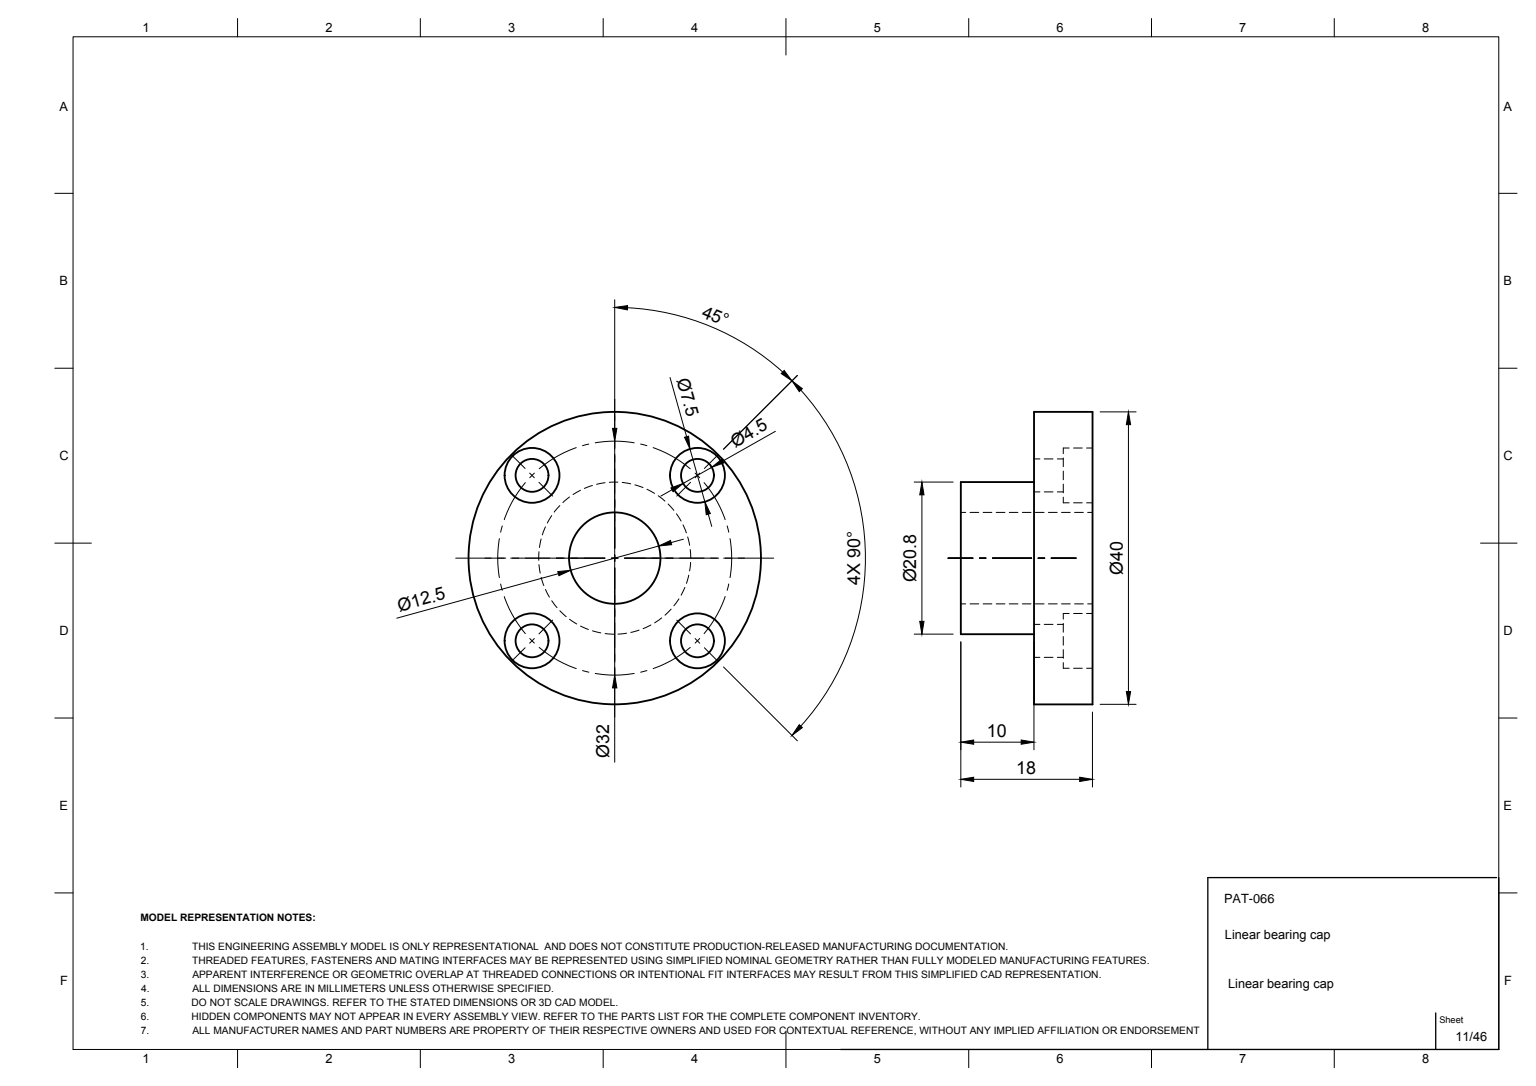
ISO-10303-21;
HEADER;
/* Generated by software containing ST-Developer
 * from STEP Tools, Inc. (www.steptools.com) 
 */

FILE_DESCRIPTION(
/* description */ ('Lever-operated bar clamp (toggle)'),
/* implementation_level */ '2;1');

FILE_NAME(
/* name */ 'Linear bearing cap.step',
/* time_stamp */ '2026-10-28T03:25:02-07:00',
/* author */ (''),
/* organization */ (''),
/* preprocessor_version */ 'ST-DEVELOPER v20.2',
/* originating_system */ 'Autodesk Translation Framework v15.17.0.0',
/* authorisation */ '');

FILE_SCHEMA (('AUTOMOTIVE_DESIGN { 1 0 10303 214 3 1 1 }'));
ENDSEC;

DATA;
#10=MECHANICAL_DESIGN_GEOMETRIC_PRESENTATION_REPRESENTATION('',(#416),#12413);
#340=SHAPE_REPRESENTATION_RELATIONSHIP('SRR','None',#12579,#378);
#378=ADVANCED_BREP_SHAPE_REPRESENTATION('',(#463),#12376);
#416=STYLED_ITEM('',(#12869),#463);
#463=MANIFOLD_SOLID_BREP('Body1',#6575);
#566=FACE_BOUND('',#1446,.T.);
#567=FACE_BOUND('',#1449,.T.);
#568=FACE_BOUND('',#1452,.T.);
#569=FACE_BOUND('',#1455,.T.);
#570=FACE_BOUND('',#1462,.T.);
#571=FACE_BOUND('',#1466,.T.);
#572=FACE_BOUND('',#1467,.T.);
#573=FACE_BOUND('',#1468,.T.);
#574=FACE_BOUND('',#1469,.T.);
#575=FACE_BOUND('',#1470,.T.);
#576=FACE_BOUND('',#1472,.T.);
#577=FACE_BOUND('',#1473,.T.);
#578=FACE_BOUND('',#1474,.T.);
#579=FACE_BOUND('',#1475,.T.);
#580=FACE_BOUND('',#1476,.T.);
#695=PLANE('',#7215);
#696=PLANE('',#7220);
#697=PLANE('',#7225);
#698=PLANE('',#7230);
#699=PLANE('',#7243);
#700=PLANE('',#7250);
#701=PLANE('',#7251);
#972=FACE_OUTER_BOUND('',#1444,.T.);
#973=FACE_OUTER_BOUND('',#1445,.T.);
#974=FACE_OUTER_BOUND('',#1447,.T.);
#975=FACE_OUTER_BOUND('',#1448,.T.);
#976=FACE_OUTER_BOUND('',#1450,.T.);
#977=FACE_OUTER_BOUND('',#1451,.T.);
#978=FACE_OUTER_BOUND('',#1453,.T.);
#979=FACE_OUTER_BOUND('',#1454,.T.);
#980=FACE_OUTER_BOUND('',#1456,.T.);
#981=FACE_OUTER_BOUND('',#1457,.T.);
#982=FACE_OUTER_BOUND('',#1458,.T.);
#983=FACE_OUTER_BOUND('',#1459,.T.);
#984=FACE_OUTER_BOUND('',#1460,.T.);
#985=FACE_OUTER_BOUND('',#1461,.T.);
#986=FACE_OUTER_BOUND('',#1463,.T.);
#987=FACE_OUTER_BOUND('',#1464,.T.);
#988=FACE_OUTER_BOUND('',#1465,.T.);
#989=FACE_OUTER_BOUND('',#1471,.T.);
#1444=EDGE_LOOP('',(#4805,#4806,#4807,#4808));
#1445=EDGE_LOOP('',(#4809));
#1446=EDGE_LOOP('',(#4810));
#1447=EDGE_LOOP('',(#4811,#4812,#4813,#4814));
#1448=EDGE_LOOP('',(#4815));
#1449=EDGE_LOOP('',(#4816));
#1450=EDGE_LOOP('',(#4817,#4818,#4819,#4820));
#1451=EDGE_LOOP('',(#4821));
#1452=EDGE_LOOP('',(#4822));
#1453=EDGE_LOOP('',(#4823,#4824,#4825,#4826));
#1454=EDGE_LOOP('',(#4827));
#1455=EDGE_LOOP('',(#4828));
#1456=EDGE_LOOP('',(#4829,#4830,#4831,#4832));
#1457=EDGE_LOOP('',(#4833,#4834,#4835,#4836));
#1458=EDGE_LOOP('',(#4837,#4838,#4839,#4840));
#1459=EDGE_LOOP('',(#4841,#4842,#4843,#4844));
#1460=EDGE_LOOP('',(#4845,#4846,#4847,#4848));
#1461=EDGE_LOOP('',(#4849));
#1462=EDGE_LOOP('',(#4850));
#1463=EDGE_LOOP('',(#4851,#4852,#4853,#4854));
#1464=EDGE_LOOP('',(#4855,#4856,#4857,#4858));
#1465=EDGE_LOOP('',(#4859));
#1466=EDGE_LOOP('',(#4860));
#1467=EDGE_LOOP('',(#4861));
#1468=EDGE_LOOP('',(#4862));
#1469=EDGE_LOOP('',(#4863));
#1470=EDGE_LOOP('',(#4864));
#1471=EDGE_LOOP('',(#4865));
#1472=EDGE_LOOP('',(#4866));
#1473=EDGE_LOOP('',(#4867));
#1474=EDGE_LOOP('',(#4868));
#1475=EDGE_LOOP('',(#4869));
#1476=EDGE_LOOP('',(#4870));
#1963=LINE('',#10462,#2404);
#1964=LINE('',#10471,#2405);
#1965=LINE('',#10480,#2406);
#1966=LINE('',#10489,#2407);
#1967=LINE('',#10497,#2408);
#1968=LINE('',#10501,#2409);
#1969=LINE('',#10505,#2410);
#1970=LINE('',#10509,#2411);
#1971=LINE('',#10514,#2412);
#1972=LINE('',#10522,#2413);
#1973=LINE('',#10527,#2414);
#2404=VECTOR('',#8356,0.375);
#2405=VECTOR('',#8367,0.375);
#2406=VECTOR('',#8378,0.375);
#2407=VECTOR('',#8389,0.375);
#2408=VECTOR('',#8400,0.225);
#2409=VECTOR('',#8405,0.225);
#2410=VECTOR('',#8410,0.225);
#2411=VECTOR('',#8415,0.225);
#2412=VECTOR('',#8420,1.04);
#2413=VECTOR('',#8431,0.625);
#2414=VECTOR('',#8436,2.);
#2813=CIRCLE('',#7213,0.375);
#2814=CIRCLE('',#7214,0.375);
#2815=CIRCLE('',#7216,0.225);
#2816=CIRCLE('',#7218,0.375);
#2817=CIRCLE('',#7219,0.375);
#2818=CIRCLE('',#7221,0.225);
#2819=CIRCLE('',#7223,0.375);
#2820=CIRCLE('',#7224,0.375);
#2821=CIRCLE('',#7226,0.225);
#2822=CIRCLE('',#7228,0.375);
#2823=CIRCLE('',#7229,0.375);
#2824=CIRCLE('',#7231,0.225);
#2825=CIRCLE('',#7233,0.225);
#2826=CIRCLE('',#7235,0.225);
#2827=CIRCLE('',#7237,0.225);
#2828=CIRCLE('',#7239,0.225);
#2829=CIRCLE('',#7241,1.04);
#2830=CIRCLE('',#7242,1.04);
#2831=CIRCLE('',#7244,0.625);
#2832=CIRCLE('',#7246,0.625);
#2833=CIRCLE('',#7248,2.);
#2834=CIRCLE('',#7249,2.);
#3202=VERTEX_POINT('',#10459);
#3203=VERTEX_POINT('',#10461);
#3204=VERTEX_POINT('',#10465);
#3205=VERTEX_POINT('',#10468);
#3206=VERTEX_POINT('',#10470);
#3207=VERTEX_POINT('',#10474);
#3208=VERTEX_POINT('',#10477);
#3209=VERTEX_POINT('',#10479);
#3210=VERTEX_POINT('',#10483);
#3211=VERTEX_POINT('',#10486);
#3212=VERTEX_POINT('',#10488);
#3213=VERTEX_POINT('',#10492);
#3214=VERTEX_POINT('',#10495);
#3215=VERTEX_POINT('',#10499);
#3216=VERTEX_POINT('',#10503);
#3217=VERTEX_POINT('',#10507);
#3218=VERTEX_POINT('',#10511);
#3219=VERTEX_POINT('',#10513);
#3220=VERTEX_POINT('',#10517);
#3221=VERTEX_POINT('',#10520);
#3222=VERTEX_POINT('',#10524);
#3223=VERTEX_POINT('',#10526);
#3807=EDGE_CURVE('',#3202,#3202,#2813,.T.);
#3808=EDGE_CURVE('',#3202,#3203,#1963,.T.);
#3809=EDGE_CURVE('',#3203,#3203,#2814,.T.);
#3810=EDGE_CURVE('',#3204,#3204,#2815,.T.);
#3811=EDGE_CURVE('',#3205,#3205,#2816,.T.);
#3812=EDGE_CURVE('',#3205,#3206,#1964,.T.);
#3813=EDGE_CURVE('',#3206,#3206,#2817,.T.);
#3814=EDGE_CURVE('',#3207,#3207,#2818,.T.);
#3815=EDGE_CURVE('',#3208,#3208,#2819,.T.);
#3816=EDGE_CURVE('',#3208,#3209,#1965,.T.);
#3817=EDGE_CURVE('',#3209,#3209,#2820,.T.);
#3818=EDGE_CURVE('',#3210,#3210,#2821,.T.);
#3819=EDGE_CURVE('',#3211,#3211,#2822,.T.);
#3820=EDGE_CURVE('',#3211,#3212,#1966,.T.);
#3821=EDGE_CURVE('',#3212,#3212,#2823,.T.);
#3822=EDGE_CURVE('',#3213,#3213,#2824,.T.);
#3823=EDGE_CURVE('',#3214,#3214,#2825,.T.);
#3824=EDGE_CURVE('',#3214,#3204,#1967,.T.);
#3825=EDGE_CURVE('',#3215,#3215,#2826,.T.);
#3826=EDGE_CURVE('',#3215,#3207,#1968,.T.);
#3827=EDGE_CURVE('',#3216,#3216,#2827,.T.);
#3828=EDGE_CURVE('',#3216,#3210,#1969,.T.);
#3829=EDGE_CURVE('',#3217,#3217,#2828,.T.);
#3830=EDGE_CURVE('',#3217,#3213,#1970,.T.);
#3831=EDGE_CURVE('',#3218,#3218,#2829,.T.);
#3832=EDGE_CURVE('',#3218,#3219,#1971,.T.);
#3833=EDGE_CURVE('',#3219,#3219,#2830,.T.);
#3834=EDGE_CURVE('',#3220,#3220,#2831,.T.);
#3835=EDGE_CURVE('',#3221,#3221,#2832,.T.);
#3836=EDGE_CURVE('',#3221,#3220,#1972,.T.);
#3837=EDGE_CURVE('',#3222,#3222,#2833,.T.);
#3838=EDGE_CURVE('',#3222,#3223,#1973,.T.);
#3839=EDGE_CURVE('',#3223,#3223,#2834,.T.);
#4805=ORIENTED_EDGE('',*,*,#3807,.F.);
#4806=ORIENTED_EDGE('',*,*,#3808,.T.);
#4807=ORIENTED_EDGE('',*,*,#3809,.F.);
#4808=ORIENTED_EDGE('',*,*,#3808,.F.);
#4809=ORIENTED_EDGE('',*,*,#3807,.T.);
#4810=ORIENTED_EDGE('',*,*,#3810,.F.);
#4811=ORIENTED_EDGE('',*,*,#3811,.F.);
#4812=ORIENTED_EDGE('',*,*,#3812,.T.);
#4813=ORIENTED_EDGE('',*,*,#3813,.F.);
#4814=ORIENTED_EDGE('',*,*,#3812,.F.);
#4815=ORIENTED_EDGE('',*,*,#3811,.T.);
#4816=ORIENTED_EDGE('',*,*,#3814,.F.);
#4817=ORIENTED_EDGE('',*,*,#3815,.F.);
#4818=ORIENTED_EDGE('',*,*,#3816,.T.);
#4819=ORIENTED_EDGE('',*,*,#3817,.F.);
#4820=ORIENTED_EDGE('',*,*,#3816,.F.);
#4821=ORIENTED_EDGE('',*,*,#3815,.T.);
#4822=ORIENTED_EDGE('',*,*,#3818,.F.);
#4823=ORIENTED_EDGE('',*,*,#3819,.F.);
#4824=ORIENTED_EDGE('',*,*,#3820,.T.);
#4825=ORIENTED_EDGE('',*,*,#3821,.F.);
#4826=ORIENTED_EDGE('',*,*,#3820,.F.);
#4827=ORIENTED_EDGE('',*,*,#3819,.T.);
#4828=ORIENTED_EDGE('',*,*,#3822,.F.);
#4829=ORIENTED_EDGE('',*,*,#3823,.F.);
#4830=ORIENTED_EDGE('',*,*,#3824,.T.);
#4831=ORIENTED_EDGE('',*,*,#3810,.T.);
#4832=ORIENTED_EDGE('',*,*,#3824,.F.);
#4833=ORIENTED_EDGE('',*,*,#3825,.F.);
#4834=ORIENTED_EDGE('',*,*,#3826,.T.);
#4835=ORIENTED_EDGE('',*,*,#3814,.T.);
#4836=ORIENTED_EDGE('',*,*,#3826,.F.);
#4837=ORIENTED_EDGE('',*,*,#3827,.F.);
#4838=ORIENTED_EDGE('',*,*,#3828,.T.);
#4839=ORIENTED_EDGE('',*,*,#3818,.T.);
#4840=ORIENTED_EDGE('',*,*,#3828,.F.);
#4841=ORIENTED_EDGE('',*,*,#3829,.F.);
#4842=ORIENTED_EDGE('',*,*,#3830,.T.);
#4843=ORIENTED_EDGE('',*,*,#3822,.T.);
#4844=ORIENTED_EDGE('',*,*,#3830,.F.);
#4845=ORIENTED_EDGE('',*,*,#3831,.F.);
#4846=ORIENTED_EDGE('',*,*,#3832,.T.);
#4847=ORIENTED_EDGE('',*,*,#3833,.T.);
#4848=ORIENTED_EDGE('',*,*,#3832,.F.);
#4849=ORIENTED_EDGE('',*,*,#3833,.F.);
#4850=ORIENTED_EDGE('',*,*,#3834,.F.);
#4851=ORIENTED_EDGE('',*,*,#3835,.F.);
#4852=ORIENTED_EDGE('',*,*,#3836,.T.);
#4853=ORIENTED_EDGE('',*,*,#3834,.T.);
#4854=ORIENTED_EDGE('',*,*,#3836,.F.);
#4855=ORIENTED_EDGE('',*,*,#3837,.F.);
#4856=ORIENTED_EDGE('',*,*,#3838,.T.);
#4857=ORIENTED_EDGE('',*,*,#3839,.T.);
#4858=ORIENTED_EDGE('',*,*,#3838,.F.);
#4859=ORIENTED_EDGE('',*,*,#3837,.T.);
#4860=ORIENTED_EDGE('',*,*,#3835,.T.);
#4861=ORIENTED_EDGE('',*,*,#3821,.T.);
#4862=ORIENTED_EDGE('',*,*,#3817,.T.);
#4863=ORIENTED_EDGE('',*,*,#3813,.T.);
#4864=ORIENTED_EDGE('',*,*,#3809,.T.);
#4865=ORIENTED_EDGE('',*,*,#3839,.F.);
#4866=ORIENTED_EDGE('',*,*,#3831,.T.);
#4867=ORIENTED_EDGE('',*,*,#3829,.T.);
#4868=ORIENTED_EDGE('',*,*,#3827,.T.);
#4869=ORIENTED_EDGE('',*,*,#3825,.T.);
#4870=ORIENTED_EDGE('',*,*,#3823,.T.);
#6073=CYLINDRICAL_SURFACE('',#7212,0.375);
#6074=CYLINDRICAL_SURFACE('',#7217,0.375);
#6075=CYLINDRICAL_SURFACE('',#7222,0.375);
#6076=CYLINDRICAL_SURFACE('',#7227,0.375);
#6077=CYLINDRICAL_SURFACE('',#7232,0.225);
#6078=CYLINDRICAL_SURFACE('',#7234,0.225);
#6079=CYLINDRICAL_SURFACE('',#7236,0.225);
#6080=CYLINDRICAL_SURFACE('',#7238,0.225);
#6081=CYLINDRICAL_SURFACE('',#7240,1.04);
#6082=CYLINDRICAL_SURFACE('',#7245,0.625);
#6083=CYLINDRICAL_SURFACE('',#7247,2.);
#6247=ADVANCED_FACE('',(#972),#6073,.F.);
#6248=ADVANCED_FACE('',(#973,#566),#695,.T.);
#6249=ADVANCED_FACE('',(#974),#6074,.F.);
#6250=ADVANCED_FACE('',(#975,#567),#696,.T.);
#6251=ADVANCED_FACE('',(#976),#6075,.F.);
#6252=ADVANCED_FACE('',(#977,#568),#697,.T.);
#6253=ADVANCED_FACE('',(#978),#6076,.F.);
#6254=ADVANCED_FACE('',(#979,#569),#698,.T.);
#6255=ADVANCED_FACE('',(#980),#6077,.F.);
#6256=ADVANCED_FACE('',(#981),#6078,.F.);
#6257=ADVANCED_FACE('',(#982),#6079,.F.);
#6258=ADVANCED_FACE('',(#983),#6080,.F.);
#6259=ADVANCED_FACE('',(#984),#6081,.T.);
#6260=ADVANCED_FACE('',(#985,#570),#699,.F.);
#6261=ADVANCED_FACE('',(#986),#6082,.F.);
#6262=ADVANCED_FACE('',(#987),#6083,.T.);
#6263=ADVANCED_FACE('',(#988,#571,#572,#573,#574,#575),#700,.T.);
#6264=ADVANCED_FACE('',(#989,#576,#577,#578,#579,#580),#701,.F.);
#6575=CLOSED_SHELL('',(#6247,#6248,#6249,#6250,#6251,#6252,#6253,#6254,
#6255,#6256,#6257,#6258,#6259,#6260,#6261,#6262,#6263,#6264));
#7211=AXIS2_PLACEMENT_3D('',#10457,#8350,#8351);
#7212=AXIS2_PLACEMENT_3D('',#10458,#8352,#8353);
#7213=AXIS2_PLACEMENT_3D('',#10460,#8354,#8355);
#7214=AXIS2_PLACEMENT_3D('',#10463,#8357,#8358);
#7215=AXIS2_PLACEMENT_3D('',#10464,#8359,#8360);
#7216=AXIS2_PLACEMENT_3D('',#10466,#8361,#8362);
#7217=AXIS2_PLACEMENT_3D('',#10467,#8363,#8364);
#7218=AXIS2_PLACEMENT_3D('',#10469,#8365,#8366);
#7219=AXIS2_PLACEMENT_3D('',#10472,#8368,#8369);
#7220=AXIS2_PLACEMENT_3D('',#10473,#8370,#8371);
#7221=AXIS2_PLACEMENT_3D('',#10475,#8372,#8373);
#7222=AXIS2_PLACEMENT_3D('',#10476,#8374,#8375);
#7223=AXIS2_PLACEMENT_3D('',#10478,#8376,#8377);
#7224=AXIS2_PLACEMENT_3D('',#10481,#8379,#8380);
#7225=AXIS2_PLACEMENT_3D('',#10482,#8381,#8382);
#7226=AXIS2_PLACEMENT_3D('',#10484,#8383,#8384);
#7227=AXIS2_PLACEMENT_3D('',#10485,#8385,#8386);
#7228=AXIS2_PLACEMENT_3D('',#10487,#8387,#8388);
#7229=AXIS2_PLACEMENT_3D('',#10490,#8390,#8391);
#7230=AXIS2_PLACEMENT_3D('',#10491,#8392,#8393);
#7231=AXIS2_PLACEMENT_3D('',#10493,#8394,#8395);
#7232=AXIS2_PLACEMENT_3D('',#10494,#8396,#8397);
#7233=AXIS2_PLACEMENT_3D('',#10496,#8398,#8399);
#7234=AXIS2_PLACEMENT_3D('',#10498,#8401,#8402);
#7235=AXIS2_PLACEMENT_3D('',#10500,#8403,#8404);
#7236=AXIS2_PLACEMENT_3D('',#10502,#8406,#8407);
#7237=AXIS2_PLACEMENT_3D('',#10504,#8408,#8409);
#7238=AXIS2_PLACEMENT_3D('',#10506,#8411,#8412);
#7239=AXIS2_PLACEMENT_3D('',#10508,#8413,#8414);
#7240=AXIS2_PLACEMENT_3D('',#10510,#8416,#8417);
#7241=AXIS2_PLACEMENT_3D('',#10512,#8418,#8419);
#7242=AXIS2_PLACEMENT_3D('',#10515,#8421,#8422);
#7243=AXIS2_PLACEMENT_3D('',#10516,#8423,#8424);
#7244=AXIS2_PLACEMENT_3D('',#10518,#8425,#8426);
#7245=AXIS2_PLACEMENT_3D('',#10519,#8427,#8428);
#7246=AXIS2_PLACEMENT_3D('',#10521,#8429,#8430);
#7247=AXIS2_PLACEMENT_3D('',#10523,#8432,#8433);
#7248=AXIS2_PLACEMENT_3D('',#10525,#8434,#8435);
#7249=AXIS2_PLACEMENT_3D('',#10528,#8437,#8438);
#7250=AXIS2_PLACEMENT_3D('',#10529,#8439,#8440);
#7251=AXIS2_PLACEMENT_3D('',#10530,#8441,#8442);
#8350=DIRECTION('axis',(0.,0.,1.));
#8351=DIRECTION('refdir',(1.,0.,0.));
#8352=DIRECTION('center_axis',(0.,0.,1.));
#8353=DIRECTION('ref_axis',(1.,0.,0.));
#8354=DIRECTION('center_axis',(0.,0.,1.));
#8355=DIRECTION('ref_axis',(1.,0.,0.));
#8356=DIRECTION('',(0.,0.,1.));
#8357=DIRECTION('center_axis',(0.,0.,-1.));
#8358=DIRECTION('ref_axis',(1.,0.,0.));
#8359=DIRECTION('center_axis',(0.,0.,1.));
#8360=DIRECTION('ref_axis',(1.,0.,0.));
#8361=DIRECTION('center_axis',(0.,0.,1.));
#8362=DIRECTION('ref_axis',(1.,0.,0.));
#8363=DIRECTION('center_axis',(0.,0.,1.));
#8364=DIRECTION('ref_axis',(1.,0.,0.));
#8365=DIRECTION('center_axis',(0.,0.,1.));
#8366=DIRECTION('ref_axis',(1.,0.,0.));
#8367=DIRECTION('',(0.,0.,1.));
#8368=DIRECTION('center_axis',(0.,0.,-1.));
#8369=DIRECTION('ref_axis',(1.,0.,0.));
#8370=DIRECTION('center_axis',(0.,0.,1.));
#8371=DIRECTION('ref_axis',(1.,0.,0.));
#8372=DIRECTION('center_axis',(0.,0.,1.));
#8373=DIRECTION('ref_axis',(1.,0.,0.));
#8374=DIRECTION('center_axis',(0.,0.,1.));
#8375=DIRECTION('ref_axis',(1.,0.,0.));
#8376=DIRECTION('center_axis',(0.,0.,1.));
#8377=DIRECTION('ref_axis',(1.,0.,0.));
#8378=DIRECTION('',(0.,0.,1.));
#8379=DIRECTION('center_axis',(0.,0.,-1.));
#8380=DIRECTION('ref_axis',(1.,0.,0.));
#8381=DIRECTION('center_axis',(0.,0.,1.));
#8382=DIRECTION('ref_axis',(1.,0.,0.));
#8383=DIRECTION('center_axis',(0.,0.,1.));
#8384=DIRECTION('ref_axis',(1.,0.,0.));
#8385=DIRECTION('center_axis',(0.,0.,1.));
#8386=DIRECTION('ref_axis',(1.,0.,0.));
#8387=DIRECTION('center_axis',(0.,0.,1.));
#8388=DIRECTION('ref_axis',(1.,0.,0.));
#8389=DIRECTION('',(0.,0.,1.));
#8390=DIRECTION('center_axis',(0.,0.,-1.));
#8391=DIRECTION('ref_axis',(1.,0.,0.));
#8392=DIRECTION('center_axis',(0.,0.,1.));
#8393=DIRECTION('ref_axis',(1.,0.,0.));
#8394=DIRECTION('center_axis',(0.,0.,1.));
#8395=DIRECTION('ref_axis',(1.,0.,0.));
#8396=DIRECTION('center_axis',(0.,0.,1.));
#8397=DIRECTION('ref_axis',(1.,0.,0.));
#8398=DIRECTION('center_axis',(0.,0.,1.));
#8399=DIRECTION('ref_axis',(1.,0.,0.));
#8400=DIRECTION('',(0.,0.,1.));
#8401=DIRECTION('center_axis',(0.,0.,1.));
#8402=DIRECTION('ref_axis',(1.,0.,0.));
#8403=DIRECTION('center_axis',(0.,0.,1.));
#8404=DIRECTION('ref_axis',(1.,0.,0.));
#8405=DIRECTION('',(0.,0.,1.));
#8406=DIRECTION('center_axis',(0.,0.,1.));
#8407=DIRECTION('ref_axis',(1.,0.,0.));
#8408=DIRECTION('center_axis',(0.,0.,1.));
#8409=DIRECTION('ref_axis',(1.,0.,0.));
#8410=DIRECTION('',(0.,0.,1.));
#8411=DIRECTION('center_axis',(0.,0.,1.));
#8412=DIRECTION('ref_axis',(1.,0.,0.));
#8413=DIRECTION('center_axis',(0.,0.,1.));
#8414=DIRECTION('ref_axis',(1.,0.,0.));
#8415=DIRECTION('',(0.,0.,1.));
#8416=DIRECTION('center_axis',(0.,0.,1.));
#8417=DIRECTION('ref_axis',(1.,0.,0.));
#8418=DIRECTION('center_axis',(0.,0.,1.));
#8419=DIRECTION('ref_axis',(1.,0.,0.));
#8420=DIRECTION('',(0.,0.,-1.));
#8421=DIRECTION('center_axis',(0.,0.,1.));
#8422=DIRECTION('ref_axis',(1.,0.,0.));
#8423=DIRECTION('center_axis',(0.,0.,1.));
#8424=DIRECTION('ref_axis',(1.,0.,0.));
#8425=DIRECTION('center_axis',(0.,0.,-1.));
#8426=DIRECTION('ref_axis',(1.,0.,0.));
#8427=DIRECTION('center_axis',(0.,0.,1.));
#8428=DIRECTION('ref_axis',(1.,0.,0.));
#8429=DIRECTION('center_axis',(0.,0.,-1.));
#8430=DIRECTION('ref_axis',(1.,0.,0.));
#8431=DIRECTION('',(0.,0.,-1.));
#8432=DIRECTION('center_axis',(0.,0.,1.));
#8433=DIRECTION('ref_axis',(1.,0.,0.));
#8434=DIRECTION('center_axis',(0.,0.,1.));
#8435=DIRECTION('ref_axis',(1.,0.,0.));
#8436=DIRECTION('',(0.,0.,-1.));
#8437=DIRECTION('center_axis',(0.,0.,1.));
#8438=DIRECTION('ref_axis',(1.,0.,0.));
#8439=DIRECTION('center_axis',(0.,0.,1.));
#8440=DIRECTION('ref_axis',(1.,0.,0.));
#8441=DIRECTION('center_axis',(0.,0.,1.));
#8442=DIRECTION('ref_axis',(1.,0.,0.));
#10457=CARTESIAN_POINT('',(0.,0.,0.));
#10458=CARTESIAN_POINT('Origin',(-1.13137084989848,-1.13137084989848,16.9));
#10459=CARTESIAN_POINT('',(-1.50637084989848,-1.13137084989848,16.9));
#10460=CARTESIAN_POINT('Origin',(-1.13137084989848,-1.13137084989848,16.9));
#10461=CARTESIAN_POINT('',(-1.50637084989848,-1.13137084989848,17.3));
#10462=CARTESIAN_POINT('',(-1.50637084989848,-1.13137084989848,16.9));
#10463=CARTESIAN_POINT('Origin',(-1.13137084989848,-1.13137084989848,17.3));
#10464=CARTESIAN_POINT('Origin',(-1.13137084989848,-1.13137084989848,16.9));
#10465=CARTESIAN_POINT('',(-1.35637084989848,-1.13137084989848,16.9));
#10466=CARTESIAN_POINT('Origin',(-1.13137084989848,-1.13137084989848,16.9));
#10467=CARTESIAN_POINT('Origin',(-1.13137084989848,1.13137084989848,16.9));
#10468=CARTESIAN_POINT('',(-1.50637084989848,1.13137084989848,16.9));
#10469=CARTESIAN_POINT('Origin',(-1.13137084989848,1.13137084989848,16.9));
#10470=CARTESIAN_POINT('',(-1.50637084989848,1.13137084989848,17.3));
#10471=CARTESIAN_POINT('',(-1.50637084989848,1.13137084989848,16.9));
#10472=CARTESIAN_POINT('Origin',(-1.13137084989848,1.13137084989848,17.3));
#10473=CARTESIAN_POINT('Origin',(-1.13137084989848,1.13137084989848,16.9));
#10474=CARTESIAN_POINT('',(-1.35637084989848,1.13137084989848,16.9));
#10475=CARTESIAN_POINT('Origin',(-1.13137084989848,1.13137084989848,16.9));
#10476=CARTESIAN_POINT('Origin',(1.13137084989848,1.13137084989848,16.9));
#10477=CARTESIAN_POINT('',(0.756370849898476,1.13137084989848,16.9));
#10478=CARTESIAN_POINT('Origin',(1.13137084989848,1.13137084989848,16.9));
#10479=CARTESIAN_POINT('',(0.756370849898476,1.13137084989848,17.3));
#10480=CARTESIAN_POINT('',(0.756370849898476,1.13137084989848,16.9));
#10481=CARTESIAN_POINT('Origin',(1.13137084989848,1.13137084989848,17.3));
#10482=CARTESIAN_POINT('Origin',(1.13137084989848,1.13137084989848,16.9));
#10483=CARTESIAN_POINT('',(0.906370849898476,1.13137084989848,16.9));
#10484=CARTESIAN_POINT('Origin',(1.13137084989848,1.13137084989848,16.9));
#10485=CARTESIAN_POINT('Origin',(1.13137084989848,-1.13137084989848,16.9));
#10486=CARTESIAN_POINT('',(0.756370849898476,-1.13137084989848,16.9));
#10487=CARTESIAN_POINT('Origin',(1.13137084989848,-1.13137084989848,16.9));
#10488=CARTESIAN_POINT('',(0.756370849898476,-1.13137084989848,17.3));
#10489=CARTESIAN_POINT('',(0.756370849898476,-1.13137084989848,16.9));
#10490=CARTESIAN_POINT('Origin',(1.13137084989848,-1.13137084989848,17.3));
#10491=CARTESIAN_POINT('Origin',(1.13137084989848,-1.13137084989848,16.9));
#10492=CARTESIAN_POINT('',(0.906370849898476,-1.13137084989848,16.9));
#10493=CARTESIAN_POINT('Origin',(1.13137084989848,-1.13137084989848,16.9));
#10494=CARTESIAN_POINT('Origin',(-1.13137084989848,-1.13137084989848,16.4));
#10495=CARTESIAN_POINT('',(-1.35637084989848,-1.13137084989848,16.5));
#10496=CARTESIAN_POINT('Origin',(-1.13137084989848,-1.13137084989848,16.5));
#10497=CARTESIAN_POINT('',(-1.35637084989848,-1.13137084989848,16.4));
#10498=CARTESIAN_POINT('Origin',(-1.13137084989848,1.13137084989848,16.4));
#10499=CARTESIAN_POINT('',(-1.35637084989848,1.13137084989848,16.5));
#10500=CARTESIAN_POINT('Origin',(-1.13137084989848,1.13137084989848,16.5));
#10501=CARTESIAN_POINT('',(-1.35637084989848,1.13137084989848,16.4));
#10502=CARTESIAN_POINT('Origin',(1.13137084989848,1.13137084989848,16.4));
#10503=CARTESIAN_POINT('',(0.906370849898476,1.13137084989848,16.5));
#10504=CARTESIAN_POINT('Origin',(1.13137084989848,1.13137084989848,16.5));
#10505=CARTESIAN_POINT('',(0.906370849898476,1.13137084989848,16.4));
#10506=CARTESIAN_POINT('Origin',(1.13137084989848,-1.13137084989848,16.4));
#10507=CARTESIAN_POINT('',(0.906370849898476,-1.13137084989848,16.5));
#10508=CARTESIAN_POINT('Origin',(1.13137084989848,-1.13137084989848,16.5));
#10509=CARTESIAN_POINT('',(0.906370849898476,-1.13137084989848,16.4));
#10510=CARTESIAN_POINT('Origin',(0.,0.,15.5));
#10511=CARTESIAN_POINT('',(-1.04,-1.27363267111325E-16,16.5));
#10512=CARTESIAN_POINT('Origin',(0.,0.,16.5));
#10513=CARTESIAN_POINT('',(-1.04,-1.27363267111325E-16,15.5));
#10514=CARTESIAN_POINT('',(-1.04,-1.27363267111325E-16,15.5));
#10515=CARTESIAN_POINT('Origin',(0.,0.,15.5));
#10516=CARTESIAN_POINT('Origin',(0.,0.,15.5));
#10517=CARTESIAN_POINT('',(-0.625,-7.65404249467096E-17,15.5));
#10518=CARTESIAN_POINT('Origin',(0.,0.,15.5));
#10519=CARTESIAN_POINT('Origin',(0.,0.,16.5));
#10520=CARTESIAN_POINT('',(-0.625,-7.65404249467096E-17,17.3));
#10521=CARTESIAN_POINT('Origin',(0.,0.,17.3));
#10522=CARTESIAN_POINT('',(-0.625,-7.65404249467096E-17,16.5));
#10523=CARTESIAN_POINT('Origin',(0.,0.,16.5));
#10524=CARTESIAN_POINT('',(-2.,-2.44929359829471E-16,17.3));
#10525=CARTESIAN_POINT('Origin',(0.,0.,17.3));
#10526=CARTESIAN_POINT('',(-2.,-2.44929359829471E-16,16.5));
#10527=CARTESIAN_POINT('',(-2.,-2.44929359829471E-16,16.5));
#10528=CARTESIAN_POINT('Origin',(0.,0.,16.5));
#10529=CARTESIAN_POINT('Origin',(0.,0.,17.3));
#10530=CARTESIAN_POINT('Origin',(0.,0.,16.5));
#12330=UNCERTAINTY_MEASURE_WITH_UNIT(LENGTH_MEASURE(0.001),#12414,
'DISTANCE_ACCURACY_VALUE',
'Maximum model space distance between geometric entities at asserted c
onnectivities');
#12367=UNCERTAINTY_MEASURE_WITH_UNIT(LENGTH_MEASURE(0.001),#12414,
'DISTANCE_ACCURACY_VALUE',
'Maximum model space distance between geometric entities at asserted c
onnectivities');
#12376=(
GEOMETRIC_REPRESENTATION_CONTEXT(3)
GLOBAL_UNCERTAINTY_ASSIGNED_CONTEXT((#12330))
GLOBAL_UNIT_ASSIGNED_CONTEXT((#12414,#12416,#12417))
REPRESENTATION_CONTEXT('','3D')
);
#12413=(
GEOMETRIC_REPRESENTATION_CONTEXT(3)
GLOBAL_UNCERTAINTY_ASSIGNED_CONTEXT((#12367))
GLOBAL_UNIT_ASSIGNED_CONTEXT((#12414,#12416,#12417))
REPRESENTATION_CONTEXT('','3D')
);
#12414=(
LENGTH_UNIT()
NAMED_UNIT(*)
SI_UNIT(.CENTI.,.METRE.)
);
#12416=(
NAMED_UNIT(*)
PLANE_ANGLE_UNIT()
SI_UNIT($,.RADIAN.)
);
#12417=(
NAMED_UNIT(*)
SI_UNIT($,.STERADIAN.)
SOLID_ANGLE_UNIT()
);
#12426=SHAPE_DEFINITION_REPRESENTATION(#12471,#12579);
#12471=PRODUCT_DEFINITION_SHAPE('',$,#12625);
#12579=SHAPE_REPRESENTATION('',(#7211),#12376);
#12616=PRODUCT_DEFINITION_CONTEXT('part definition',#12753,'design');
#12625=PRODUCT_DEFINITION('Linear bearing cap','Linear bearing cap',#12670,
#12616);
#12670=PRODUCT_DEFINITION_FORMATION('',$,#12763);
#12753=APPLICATION_CONTEXT(
'Core Data for Automotive Mechanical Design Process');
#12754=PRODUCT_CONTEXT('part definition',#12753,'mechanical');
#12763=PRODUCT('Linear bearing cap','Linear bearing cap',
'Linear bearing cap',(#12754));
#12863=COLOUR_RGB('Grey',0.48,0.52,0.57);
#12864=FILL_AREA_STYLE_COLOUR('',#12863);
#12865=FILL_AREA_STYLE('',(#12864));
#12866=SURFACE_STYLE_FILL_AREA(#12865);
#12867=SURFACE_SIDE_STYLE('',(#12866));
#12868=SURFACE_STYLE_USAGE(.BOTH.,#12867);
#12869=PRESENTATION_STYLE_ASSIGNMENT((#12868));
ENDSEC;
END-ISO-10303-21;
